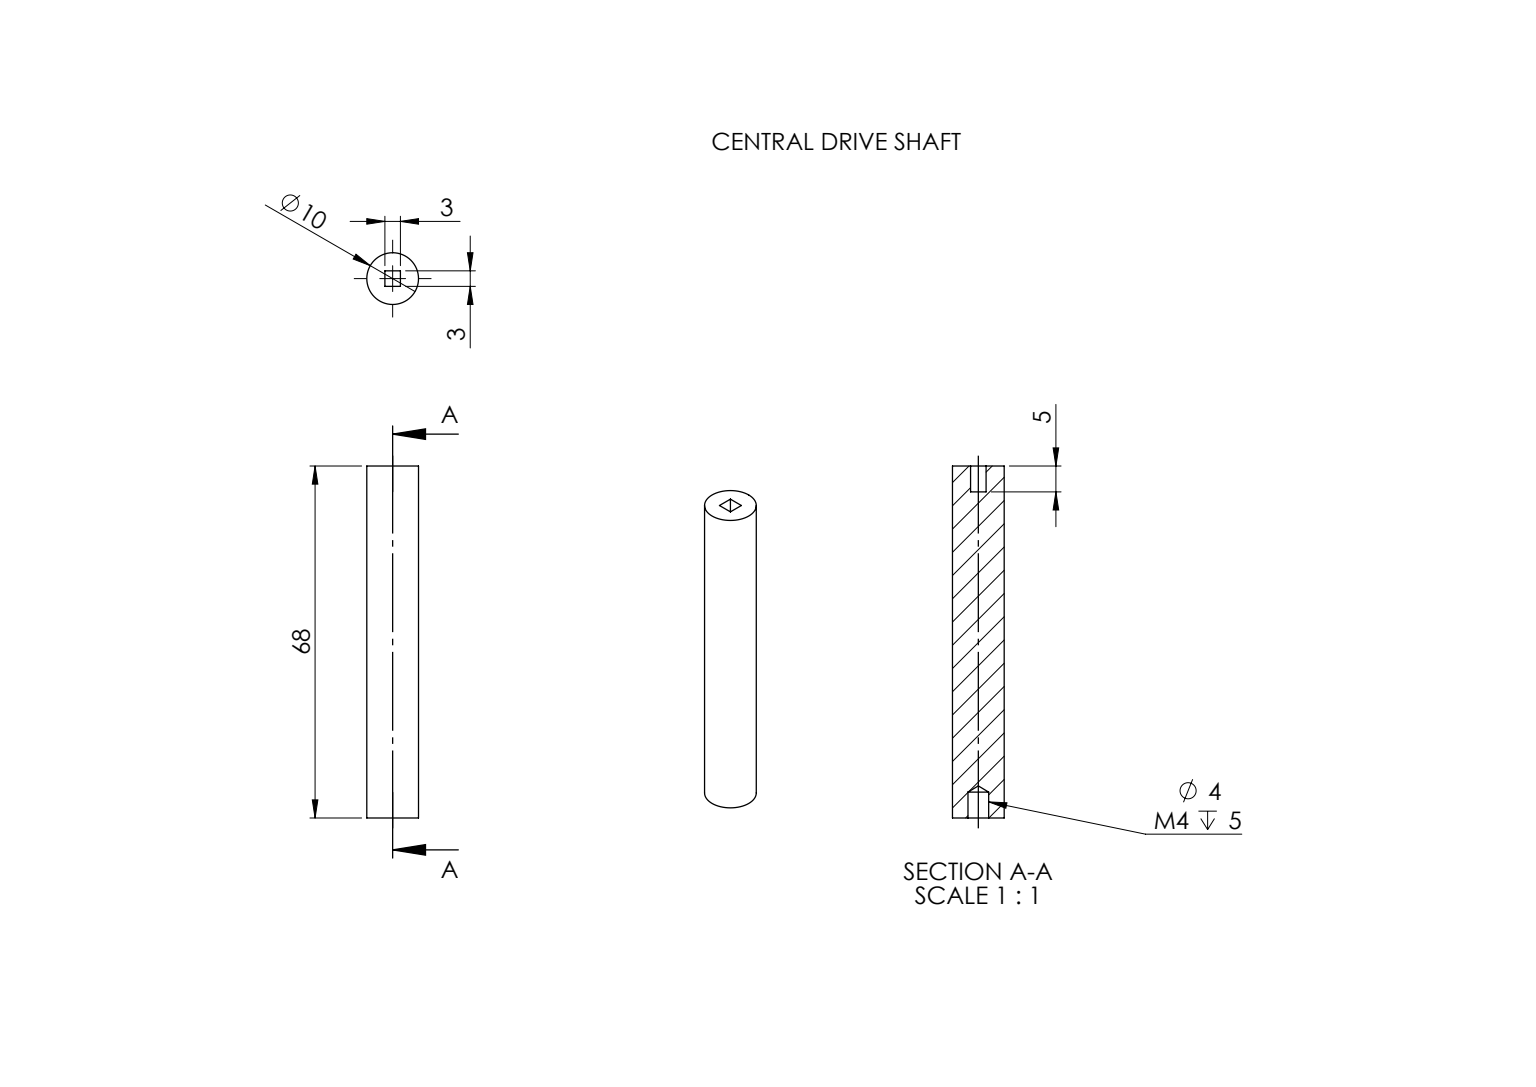
ISO-10303-21;
HEADER;
FILE_DESCRIPTION (('STEP AP214'),
    '1' );
FILE_NAME ('Central Drive Shaft.step',
    '2026-10-04T07:23:31',
    ( '' ),
    ( '' ),
    'SwSTEP 2.0',
    'SolidWorks 2026',
    '' );
FILE_SCHEMA (( 'AUTOMOTIVE_DESIGN' ));
ENDSEC;

DATA;
#2=VERTEX_POINT ( 'NONE', #10191 ) ;
#44=DIRECTION ( 'NONE',  ( 0.000000000000000000, 0.000000000000000000, -1.000000000000000000 ) ) ;
#47=ORIENTED_EDGE ( 'NONE', *, *, #865, .T. ) ;
#60=CARTESIAN_POINT ( 'NONE',  ( -1.500000000000000444, 83.00000000000000000, -1.500000000000000222 ) ) ;
#114=DIRECTION ( 'NONE',  ( 1.000000000000000000, 0.000000000000000000, -0.000000000000000000 ) ) ;
#146=DIRECTION ( 'NONE',  ( -0.000000000000000000, -1.000000000000000000, -0.000000000000000000 ) ) ;
#223=CARTESIAN_POINT ( 'NONE',  ( 0.000000000000000000, 25.00000000000000355, -2.000000000000000000 ) ) ;
#266=DIRECTION ( 'NONE',  ( 0.000000000000000000, 0.000000000000000000, -1.000000000000000000 ) ) ;
#348=DIRECTION ( 'NONE',  ( 0.000000000000000000, 0.000000000000000000, -1.000000000000000000 ) ) ;
#352=( LENGTH_UNIT ( ) NAMED_UNIT ( * ) SI_UNIT ( .MILLI., .METRE. ) );
#356=PLANE ( 'NONE',  #3904 ) ;
#359=ORIENTED_EDGE ( 'NONE', *, *, #8815, .F. ) ;
#393=ORIENTED_EDGE ( 'NONE', *, *, #10575, .T. ) ;
#405=CIRCLE ( 'NONE', #9386, 2.000000000000000000 ) ;
#454=CARTESIAN_POINT ( 'NONE',  ( 0.000000000000000000, 88.00000000000001421, 0.000000000000000000 ) ) ;
#460=CARTESIAN_POINT ( 'NONE',  ( 0.000000000000000000, 88.00000000000001421, -4.999999999999997335 ) ) ;
#485=MECHANICAL_DESIGN_GEOMETRIC_PRESENTATION_REPRESENTATION('',(#10900),#6489);
#492=VERTEX_POINT ( 'NONE', #223 ) ;
#536=DIRECTION ( 'NONE',  ( 0.000000000000000000, 1.000000000000000000, 0.000000000000000000 ) ) ;
#537=ORIENTED_EDGE ( 'NONE', *, *, #3535, .F. ) ;
#559=DIRECTION ( 'NONE',  ( 1.445602896647339163E-16, 0.000000000000000000, 1.000000000000000000 ) ) ;
#632=EDGE_LOOP ( 'NONE', ( #359, #6659, #4247, #3379 ) ) ;
#649=LINE ( 'NONE', #7380, #8128 ) ;
#650=SURFACE_STYLE_USAGE ( .BOTH. , #5631 ) ;
#693=CARTESIAN_POINT ( 'NONE',  ( -1.500000000000000444, 83.00000000000000000, -1.500000000000000222 ) ) ;
#753=CARTESIAN_POINT ( 'NONE',  ( 0.000000000000000000, 20.00000000000000355, 0.000000000000000000 ) ) ;
#771=VECTOR ( 'NONE', #10871, 1000.000000000000000 ) ;
#785=SURFACE_STYLE_FILL_AREA ( #5806 ) ;
#787=CARTESIAN_POINT ( 'NONE',  ( 0.000000000000000000, 26.20172123805511788, 0.000000000000000000 ) ) ;
#795=VERTEX_POINT ( 'NONE', #460 ) ;
#859=VERTEX_POINT ( 'NONE', #787 ) ;
#865=EDGE_CURVE ( 'NONE', #4894, #10263, #9114, .T. ) ;
#872=PLANE ( 'NONE',  #1414 ) ;
#1039=EDGE_LOOP ( 'NONE', ( #7017, #6117, #1492, #5769 ) ) ;
#1055=LINE ( 'NONE', #10332, #4311 ) ;
#1056=DIRECTION ( 'NONE',  ( -0.000000000000000000, -1.000000000000000000, -0.000000000000000000 ) ) ;
#1156=ORIENTED_EDGE ( 'NONE', *, *, #1512, .F. ) ;
#1161=CYLINDRICAL_SURFACE ( 'NONE', #5135, 2.000000000000000000 ) ;
#1178=ORIENTED_EDGE ( 'NONE', *, *, #2398, .T. ) ;
#1228=LINE ( 'NONE', #7862, #1419 ) ;
#1356=DIRECTION ( 'NONE',  ( 0.000000000000000000, 0.000000000000000000, -1.000000000000000000 ) ) ;
#1360=STYLED_ITEM ( 'NONE', ( #2425 ), #9406 ) ;
#1365=VECTOR ( 'NONE', #5254, 1000.000000000000000 ) ;
#1414=AXIS2_PLACEMENT_3D ( 'NONE', #7498, #1757, #3275 ) ;
#1419=VECTOR ( 'NONE', #2096, 1000.000000000000000 ) ;
#1443=ORIENTED_EDGE ( 'NONE', *, *, #6772, .F. ) ;
#1448=AXIS2_PLACEMENT_3D ( 'NONE', #4540, #3796, #1356 ) ;
#1468=AXIS2_PLACEMENT_3D ( 'NONE', #5195, #2673, #1693 ) ;
#1492=ORIENTED_EDGE ( 'NONE', *, *, #2347, .T. ) ;
#1499=SHAPE_REPRESENTATION_RELATIONSHIP ( 'NONE' , 'NONE' ,  #2382, #9406 ) ;
#1500=DIRECTION ( 'NONE',  ( -0.000000000000000000, -1.000000000000000000, -0.000000000000000000 ) ) ;
#1512=EDGE_CURVE ( 'NONE', #7692, #795, #8292, .T. ) ;
#1521=DIRECTION ( 'NONE',  ( 0.000000000000000000, -0.000000000000000000, 1.000000000000000000 ) ) ;
#1554=COLOUR_RGB ( '', 0.08235294, 0.09019608, 0.10196078) ;
#1588=ADVANCED_FACE ( 'NONE', ( #6010 ), #1161, .F. ) ;
#1649=PRODUCT_CONTEXT ( 'NONE', #4853, 'mechanical' ) ;
#1654=CONICAL_SURFACE ( 'NONE', #4677, 2.000000000000000000, 1.029744258676657198 ) ;
#1693=DIRECTION ( 'NONE',  ( 0.000000000000000000, 0.000000000000000000, -1.000000000000000000 ) ) ;
#1705=ORIENTED_EDGE ( 'NONE', *, *, #4329, .F. ) ;
#1712=( NAMED_UNIT ( * ) PLANE_ANGLE_UNIT ( ) SI_UNIT ( $, .RADIAN. ) );
#1719=COLOUR_RGB ( '', 0.08235294, 0.09019608, 0.10196078) ;
#1725=UNCERTAINTY_MEASURE_WITH_UNIT (LENGTH_MEASURE( 1.000000000000000082E-05 ), #9113, 'distance_accuracy_value', 'NONE');
#1739=ORIENTED_EDGE ( 'NONE', *, *, #5885, .T. ) ;
#1744=DIRECTION ( 'NONE',  ( 0.000000000000000000, 0.000000000000000000, -1.000000000000000000 ) ) ;
#1757=DIRECTION ( 'NONE',  ( -0.000000000000000000, 0.000000000000000000, 1.000000000000000000 ) ) ;
#1759=LINE ( 'NONE', #6132, #1365 ) ;
#1781=VECTOR ( 'NONE', #8968, 1000.000000000000000 ) ;
#1819=FACE_OUTER_BOUND ( 'NONE', #7522, .T. ) ;
#1843=VERTEX_POINT ( 'NONE', #7167 ) ;
#1904=CARTESIAN_POINT ( 'NONE',  ( 0.000000000000000000, 0.000000000000000000, 0.000000000000000000 ) ) ;
#1953=PRODUCT_DEFINITION_SHAPE ( 'NONE', 'NONE',  #6924 ) ;
#1990=LINE ( 'NONE', #2225, #1781 ) ;
#2005=DIRECTION ( 'NONE',  ( -0.000000000000000000, -0.000000000000000000, -1.000000000000000000 ) ) ;
#2007=CARTESIAN_POINT ( 'NONE',  ( -1.500000000000000444, 83.00000000000000000, 1.499999999999999778 ) ) ;
#2016=ORIENTED_EDGE ( 'NONE', *, *, #3973, .F. ) ;
#2018=ADVANCED_FACE ( 'NONE', ( #4526, #8756 ), #356, .T. ) ;
#2096=DIRECTION ( 'NONE',  ( 1.000000000000000000, 0.000000000000000000, 0.000000000000000000 ) ) ;
#2148=LINE ( 'NONE', #8679, #6194 ) ;
#2201=EDGE_CURVE ( 'NONE', #859, #2, #10622, .T. ) ;
#2225=CARTESIAN_POINT ( 'NONE',  ( 0.000000000000000000, 88.00000000000001421, -4.999999999999997335 ) ) ;
#2228=FACE_OUTER_BOUND ( 'NONE', #6950, .T. ) ;
#2245=SURFACE_STYLE_FILL_AREA ( #9813 ) ;
#2268=CARTESIAN_POINT ( 'NONE',  ( -1.500000000000000444, 88.00000000000001421, -1.500000000000000222 ) ) ;
#2320=FILL_AREA_STYLE_COLOUR ( '', #1554 ) ;
#2332=ORIENTED_EDGE ( 'NONE', *, *, #3800, .T. ) ;
#2347=EDGE_CURVE ( 'NONE', #6423, #4034, #2479, .T. ) ;
#2382=SHAPE_REPRESENTATION ( 'Central Drive Shaft', ( #7040 ), #8612 ) ;
#2398=EDGE_CURVE ( 'NONE', #1843, #6119, #8817, .T. ) ;
#2425=PRESENTATION_STYLE_ASSIGNMENT (( #9885 ) ) ;
#2435=CYLINDRICAL_SURFACE ( 'NONE', #8843, 4.999999999999997335 ) ;
#2460=CARTESIAN_POINT ( 'NONE',  ( 1.500000000000000000, 83.00000000000000000, 1.500000000000000000 ) ) ;
#2479=LINE ( 'NONE', #10002, #10939 ) ;
#2497=CONICAL_SURFACE ( 'NONE', #4996, 2.000000000000000000, 1.029744258676657198 ) ;
#2503=CARTESIAN_POINT ( 'NONE',  ( 0.000000000000000000, 88.00000000000001421, 0.000000000000000000 ) ) ;
#2519=FACE_OUTER_BOUND ( 'NONE', #3141, .T. ) ;
#2521=ADVANCED_FACE ( 'NONE', ( #3254 ), #10013, .T. ) ;
#2629=VECTOR ( 'NONE', #9256, 1000.000000000000000 ) ;
#2639=FACE_OUTER_BOUND ( 'NONE', #8178, .T. ) ;
#2673=DIRECTION ( 'NONE',  ( -0.000000000000000000, -1.000000000000000000, -0.000000000000000000 ) ) ;
#2736=ORIENTED_EDGE ( 'NONE', *, *, #6328, .T. ) ;
#2857=CIRCLE ( 'NONE', #4995, 4.999999999999997335 ) ;
#2884=DIRECTION ( 'NONE',  ( 0.000000000000000000, -0.000000000000000000, -1.000000000000000000 ) ) ;
#3114=CARTESIAN_POINT ( 'NONE',  ( -1.500000000000000444, 83.00000000000000000, 1.499999999999999778 ) ) ;
#3122=VECTOR ( 'NONE', #9223, 1000.000000000000000 ) ;
#3127=ORIENTED_EDGE ( 'NONE', *, *, #9759, .F. ) ;
#3141=EDGE_LOOP ( 'NONE', ( #6644, #3675, #8996 ) ) ;
#3201=DIRECTION ( 'NONE',  ( 0.000000000000000000, 0.000000000000000000, -1.000000000000000000 ) ) ;
#3254=FACE_OUTER_BOUND ( 'NONE', #632, .T. ) ;
#3275=DIRECTION ( 'NONE',  ( 1.000000000000000000, 0.000000000000000000, 0.000000000000000000 ) ) ;
#3306=FACE_OUTER_BOUND ( 'NONE', #4013, .T. ) ;
#3320=EDGE_CURVE ( 'NONE', #9769, #4894, #649, .T. ) ;
#3341=LINE ( 'NONE', #5907, #2629 ) ;
#3359=VECTOR ( 'NONE', #3900, 1000.000000000000000 ) ;
#3379=ORIENTED_EDGE ( 'NONE', *, *, #8473, .T. ) ;
#3402=ADVANCED_FACE ( 'NONE', ( #9376, #6675 ), #5136, .F. ) ;
#3416=ADVANCED_FACE ( 'NONE', ( #1819 ), #872, .T. ) ;
#3418=PLANE ( 'NONE',  #9594 ) ;
#3431=DIRECTION ( 'NONE',  ( 0.000000000000000000, 0.000000000000000000, 1.000000000000000000 ) ) ;
#3445=FACE_OUTER_BOUND ( 'NONE', #8136, .T. ) ;
#3448=CARTESIAN_POINT ( 'NONE',  ( 0.000000000000000000, 20.00000000000000355, 0.000000000000000000 ) ) ;
#3531=EDGE_LOOP ( 'NONE', ( #9699, #10736 ) ) ;
#3535=EDGE_CURVE ( 'NONE', #795, #4001, #1990, .T. ) ;
#3549=AXIS2_PLACEMENT_3D ( 'NONE', #5110, #6714, #7420 ) ;
#3621=LINE ( 'NONE', #4346, #5871 ) ;
#3627=DIRECTION ( 'NONE',  ( -0.000000000000000000, -1.000000000000000000, -0.000000000000000000 ) ) ;
#3640=ADVANCED_FACE ( 'NONE', ( #3306 ), #2435, .T. ) ;
#3641=DIRECTION ( 'NONE',  ( 0.000000000000000000, -1.000000000000000000, 0.000000000000000000 ) ) ;
#3674=ORIENTED_EDGE ( 'NONE', *, *, #10458, .F. ) ;
#3675=ORIENTED_EDGE ( 'NONE', *, *, #2201, .T. ) ;
#3774=VERTEX_POINT ( 'NONE', #9994 ) ;
#3796=DIRECTION ( 'NONE',  ( -0.000000000000000000, -1.000000000000000000, -0.000000000000000000 ) ) ;
#3800=EDGE_CURVE ( 'NONE', #3774, #10263, #4988, .T. ) ;
#3811=DIRECTION ( 'NONE',  ( 1.445602896647339163E-16, 0.000000000000000000, 1.000000000000000000 ) ) ;
#3900=DIRECTION ( 'NONE',  ( -0.000000000000000000, 1.000000000000000000, -0.000000000000000000 ) ) ;
#3904=AXIS2_PLACEMENT_3D ( 'NONE', #7105, #10470, #2884 ) ;
#3947=EDGE_LOOP ( 'NONE', ( #9642, #1156 ) ) ;
#3951=EDGE_LOOP ( 'NONE', ( #5906, #4563 ) ) ;
#3973=EDGE_CURVE ( 'NONE', #8246, #3774, #1228, .T. ) ;
#3983=CARTESIAN_POINT ( 'NONE',  ( 6.123233995736763324E-16, 20.00000000000000355, 4.999999999999997335 ) ) ;
#4001=VERTEX_POINT ( 'NONE', #7184 ) ;
#4013=EDGE_LOOP ( 'NONE', ( #1739, #8966, #1443, #537 ) ) ;
#4024=EDGE_CURVE ( 'NONE', #3774, #6423, #2148, .T. ) ;
#4034=VERTEX_POINT ( 'NONE', #2007 ) ;
#4158=CARTESIAN_POINT ( 'NONE',  ( 1.500000000000000000, 88.00000000000001421, 1.500000000000000000 ) ) ;
#4159=DIRECTION ( 'NONE',  ( -1.000000000000000000, -0.000000000000000000, -7.228014483236695816E-17 ) ) ;
#4190=SHAPE_DEFINITION_REPRESENTATION ( #1953, #2382 ) ;
#4229=VECTOR ( 'NONE', #8226, 1000.000000000000000 ) ;
#4247=ORIENTED_EDGE ( 'NONE', *, *, #4024, .T. ) ;
#4263=DIRECTION ( 'NONE',  ( -0.000000000000000000, -1.000000000000000000, -0.000000000000000000 ) ) ;
#4279=VECTOR ( 'NONE', #2005, 1000.000000000000000 ) ;
#4311=VECTOR ( 'NONE', #3641, 1000.000000000000000 ) ;
#4329=EDGE_CURVE ( 'NONE', #492, #6119, #3341, .T. ) ;
#4346=CARTESIAN_POINT ( 'NONE',  ( 2.449293598294706414E-16, 20.00000000000000355, 2.000000000000000000 ) ) ;
#4526=FACE_BOUND ( 'NONE', #3531, .T. ) ;
#4540=CARTESIAN_POINT ( 'NONE',  ( 0.000000000000000000, 20.00000000000000355, 0.000000000000000000 ) ) ;
#4563=ORIENTED_EDGE ( 'NONE', *, *, #8479, .T. ) ;
#4597=FACE_OUTER_BOUND ( 'NONE', #1039, .T. ) ;
#4606=AXIS2_PLACEMENT_3D ( 'NONE', #6774, #6652, #5062 ) ;
#4630=CIRCLE ( 'NONE', #3549, 4.999999999999997335 ) ;
#4677=AXIS2_PLACEMENT_3D ( 'NONE', #10800, #8194, #6444 ) ;
#4693=CARTESIAN_POINT ( 'NONE',  ( 0.000000000000000000, 25.00000000000000355, 0.000000000000000000 ) ) ;
#4848=CARTESIAN_POINT ( 'NONE',  ( 1.500000000000000000, 83.00000000000000000, 1.500000000000000000 ) ) ;
#4853=APPLICATION_CONTEXT ( 'automotive_design' ) ;
#4865=DIRECTION ( 'NONE',  ( -0.000000000000000000, -0.000000000000000000, -1.000000000000000000 ) ) ;
#4867=ADVANCED_FACE ( 'NONE', ( #3445 ), #5193, .T. ) ;
#4881=CARTESIAN_POINT ( 'NONE',  ( 0.000000000000000000, 20.00000000000000355, 0.000000000000000000 ) ) ;
#4893=ORIENTED_EDGE ( 'NONE', *, *, #5065, .T. ) ;
#4894=VERTEX_POINT ( 'NONE', #6070 ) ;
#4902=LINE ( 'NONE', #693, #771 ) ;
#4924=ORIENTED_EDGE ( 'NONE', *, *, #9689, .T. ) ;
#4948=AXIS2_PLACEMENT_3D ( 'NONE', #4881, #1500, #10784 ) ;
#4988=LINE ( 'NONE', #6698, #4229 ) ;
#4995=AXIS2_PLACEMENT_3D ( 'NONE', #753, #6723, #1744 ) ;
#4996=AXIS2_PLACEMENT_3D ( 'NONE', #5909, #1056, #44 ) ;
#5043=ORIENTED_EDGE ( 'NONE', *, *, #8094, .T. ) ;
#5053=ORIENTED_EDGE ( 'NONE', *, *, #8479, .F. ) ;
#5062=DIRECTION ( 'NONE',  ( 1.445602896647339163E-16, 0.000000000000000000, 1.000000000000000000 ) ) ;
#5065=EDGE_CURVE ( 'NONE', #859, #492, #9026, .T. ) ;
#5071=ADVANCED_FACE ( 'NONE', ( #2228 ), #1654, .F. ) ;
#5078=EDGE_LOOP ( 'NONE', ( #3127, #8413, #1178, #1705 ) ) ;
#5110=CARTESIAN_POINT ( 'NONE',  ( 0.000000000000000000, 20.00000000000000355, 0.000000000000000000 ) ) ;
#5135=AXIS2_PLACEMENT_3D ( 'NONE', #3448, #3627, #266 ) ;
#5136=PLANE ( 'NONE',  #6727 ) ;
#5193=CYLINDRICAL_SURFACE ( 'NONE', #7650, 4.999999999999997335 ) ;
#5195=CARTESIAN_POINT ( 'NONE',  ( 0.000000000000000000, 25.00000000000000355, 0.000000000000000000 ) ) ;
#5254=DIRECTION ( 'NONE',  ( -1.000000000000000000, -0.000000000000000000, -7.228014483236695816E-17 ) ) ;
#5419=DIRECTION ( 'NONE',  ( 0.000000000000000000, 0.000000000000000000, -1.000000000000000000 ) ) ;
#5519=ADVANCED_FACE ( 'NONE', ( #2519 ), #2497, .F. ) ;
#5601=MECHANICAL_DESIGN_GEOMETRIC_PRESENTATION_REPRESENTATION('',(#1360),#8410);
#5606=UNCERTAINTY_MEASURE_WITH_UNIT (LENGTH_MEASURE( 1.000000000000000082E-05 ), #352, 'distance_accuracy_value', 'NONE');
#5631=SURFACE_SIDE_STYLE ('',( #2245 ) ) ;
#5749=ORIENTED_EDGE ( 'NONE', *, *, #3973, .T. ) ;
#5769=ORIENTED_EDGE ( 'NONE', *, *, #10458, .T. ) ;
#5806=FILL_AREA_STYLE ('',( #2320 ) ) ;
#5818=ORIENTED_EDGE ( 'NONE', *, *, #2347, .F. ) ;
#5869=CARTESIAN_POINT ( 'NONE',  ( 2.449293598294706414E-16, 25.00000000000000355, 2.000000000000000000 ) ) ;
#5870=EDGE_CURVE ( 'NONE', #492, #2, #10108, .T. ) ;
#5871=VECTOR ( 'NONE', #146, 1000.000000000000000 ) ;
#5885=EDGE_CURVE ( 'NONE', #795, #7692, #9412, .T. ) ;
#5903=DIRECTION ( 'NONE',  ( 0.000000000000000000, -1.000000000000000000, 0.000000000000000000 ) ) ;
#5906=ORIENTED_EDGE ( 'NONE', *, *, #6772, .T. ) ;
#5907=CARTESIAN_POINT ( 'NONE',  ( 0.000000000000000000, 20.00000000000000355, -2.000000000000000000 ) ) ;
#5909=CARTESIAN_POINT ( 'NONE',  ( 0.000000000000000000, 25.00000000000000355, 0.000000000000000000 ) ) ;
#5925=DIRECTION ( 'NONE',  ( 1.049727191138620421E-16, -0.5150380749100518241, 0.8571673007021137769 ) ) ;
#6007=DIRECTION ( 'NONE',  ( 0.000000000000000000, -1.000000000000000000, 0.000000000000000000 ) ) ;
#6010=FACE_OUTER_BOUND ( 'NONE', #5078, .T. ) ;
#6070=CARTESIAN_POINT ( 'NONE',  ( -1.500000000000000444, 88.00000000000001421, -1.500000000000000222 ) ) ;
#6104=PRODUCT ( 'Central Drive Shaft', 'Central Drive Shaft', '', ( #1649 ) ) ;
#6117=ORIENTED_EDGE ( 'NONE', *, *, #8473, .F. ) ;
#6119=VERTEX_POINT ( 'NONE', #7680 ) ;
#6131=ORIENTED_EDGE ( 'NONE', *, *, #5870, .F. ) ;
#6132=CARTESIAN_POINT ( 'NONE',  ( -1.500000000000000444, 88.00000000000001421, 1.499999999999999778 ) ) ;
#6194=VECTOR ( 'NONE', #3811, 1000.000000000000000 ) ;
#6239=CARTESIAN_POINT ( 'NONE',  ( -1.500000000000000444, 83.00000000000000000, -1.500000000000000222 ) ) ;
#6253=CARTESIAN_POINT ( 'NONE',  ( -1.500000000000000444, 83.00000000000000000, 1.499999999999999778 ) ) ;
#6304=LINE ( 'NONE', #10446, #4279 ) ;
#6328=EDGE_CURVE ( 'NONE', #4034, #8246, #6304, .T. ) ;
#6379=( NAMED_UNIT ( * ) PLANE_ANGLE_UNIT ( ) SI_UNIT ( $, .RADIAN. ) );
#6408=CARTESIAN_POINT ( 'NONE',  ( 0.000000000000000000, 83.00000000000000000, 0.000000000000000000 ) ) ;
#6423=VERTEX_POINT ( 'NONE', #2460 ) ;
#6444=DIRECTION ( 'NONE',  ( 0.000000000000000000, 0.000000000000000000, -1.000000000000000000 ) ) ;
#6461=FILL_AREA_STYLE_COLOUR ( '', #1719 ) ;
#6489=( GEOMETRIC_REPRESENTATION_CONTEXT ( 3 ) GLOBAL_UNCERTAINTY_ASSIGNED_CONTEXT ( ( #9021 ) ) GLOBAL_UNIT_ASSIGNED_CONTEXT ( ( #10704, #10758, #10266 ) ) REPRESENTATION_CONTEXT ( 'NONE', 'WORKASPACE' ) );
#6517=PRODUCT_DEFINITION_FORMATION_WITH_SPECIFIED_SOURCE ( 'ANY', '', #6104, .NOT_KNOWN. ) ;
#6539=AXIS2_PLACEMENT_3D ( 'NONE', #454, #9524, #348 ) ;
#6563=AXIS2_PLACEMENT_3D ( 'NONE', #10169, #4263, #5419 ) ;
#6578=ORIENTED_EDGE ( 'NONE', *, *, #3320, .T. ) ;
#6644=ORIENTED_EDGE ( 'NONE', *, *, #5065, .F. ) ;
#6652=DIRECTION ( 'NONE',  ( -1.000000000000000000, 0.000000000000000000, 1.445602896647339163E-16 ) ) ;
#6659=ORIENTED_EDGE ( 'NONE', *, *, #3800, .F. ) ;
#6675=FACE_BOUND ( 'NONE', #7451, .T. ) ;
#6676=DIRECTION ( 'NONE',  ( -0.000000000000000000, 1.000000000000000000, -0.000000000000000000 ) ) ;
#6698=CARTESIAN_POINT ( 'NONE',  ( 1.499999999999999556, 83.00000000000000000, -1.500000000000000222 ) ) ;
#6714=DIRECTION ( 'NONE',  ( 0.000000000000000000, -1.000000000000000000, 0.000000000000000000 ) ) ;
#6723=DIRECTION ( 'NONE',  ( 0.000000000000000000, -1.000000000000000000, 0.000000000000000000 ) ) ;
#6727=AXIS2_PLACEMENT_3D ( 'NONE', #8486, #5903, #9252 ) ;
#6750=ORIENTED_EDGE ( 'NONE', *, *, #5870, .T. ) ;
#6755=CIRCLE ( 'NONE', #1448, 2.000000000000000000 ) ;
#6771=AXIS2_PLACEMENT_3D ( 'NONE', #2503, #7716, #6962 ) ;
#6772=EDGE_CURVE ( 'NONE', #4001, #7375, #2857, .T. ) ;
#6774=CARTESIAN_POINT ( 'NONE',  ( 1.499999999999999556, 83.00000000000000000, -1.500000000000000222 ) ) ;
#6836=CARTESIAN_POINT ( 'NONE',  ( 0.000000000000000000, 88.00000000000001421, 0.000000000000000000 ) ) ;
#6899=DIRECTION ( 'NONE',  ( 0.000000000000000000, 0.000000000000000000, -1.000000000000000000 ) ) ;
#6924=PRODUCT_DEFINITION ( 'UNKNOWN', '', #6517, #8802 ) ;
#6949=EDGE_CURVE ( 'NONE', #2, #1843, #3621, .T. ) ;
#6950=EDGE_LOOP ( 'NONE', ( #10094, #4893, #6750 ) ) ;
#6962=DIRECTION ( 'NONE',  ( 0.000000000000000000, 0.000000000000000000, -1.000000000000000000 ) ) ;
#6970=VECTOR ( 'NONE', #8240, 1000.000000000000114 ) ;
#6988=ORIENTED_EDGE ( 'NONE', *, *, #1512, .T. ) ;
#6989=ORIENTED_EDGE ( 'NONE', *, *, #6328, .F. ) ;
#7017=ORIENTED_EDGE ( 'NONE', *, *, #10575, .F. ) ;
#7040=AXIS2_PLACEMENT_3D ( 'NONE', #1904, #3431, #7048 ) ;
#7048=DIRECTION ( 'NONE',  ( 1.000000000000000000, 0.000000000000000000, 0.000000000000000000 ) ) ;
#7071=ORIENTED_EDGE ( 'NONE', *, *, #6949, .F. ) ;
#7105=CARTESIAN_POINT ( 'NONE',  ( 0.000000000000000000, 20.00000000000000355, 0.000000000000000000 ) ) ;
#7130=AXIS2_PLACEMENT_3D ( 'NONE', #6253, #9557, #7791 ) ;
#7167=CARTESIAN_POINT ( 'NONE',  ( 2.449293598294706414E-16, 20.00000000000000355, 2.000000000000000000 ) ) ;
#7184=CARTESIAN_POINT ( 'NONE',  ( 0.000000000000000000, 20.00000000000000355, -4.999999999999997335 ) ) ;
#7196=ADVANCED_FACE ( 'NONE', ( #2639 ), #3418, .T. ) ;
#7322=FACE_OUTER_BOUND ( 'NONE', #8137, .T. ) ;
#7375=VERTEX_POINT ( 'NONE', #3983 ) ;
#7380=CARTESIAN_POINT ( 'NONE',  ( -1.500000000000000444, 88.00000000000001421, -1.500000000000000222 ) ) ;
#7414=DIRECTION ( 'NONE',  ( 0.000000000000000000, -1.000000000000000000, 0.000000000000000000 ) ) ;
#7420=DIRECTION ( 'NONE',  ( 0.000000000000000000, 0.000000000000000000, -1.000000000000000000 ) ) ;
#7451=EDGE_LOOP ( 'NONE', ( #10021, #393, #6578, #47 ) ) ;
#7498=CARTESIAN_POINT ( 'NONE',  ( -1.500000000000000444, 83.00000000000000000, -1.500000000000000222 ) ) ;
#7522=EDGE_LOOP ( 'NONE', ( #8899, #9738, #5749, #2332 ) ) ;
#7567=DIRECTION ( 'NONE',  ( -0.000000000000000000, 0.000000000000000000, -1.000000000000000000 ) ) ;
#7650=AXIS2_PLACEMENT_3D ( 'NONE', #6836, #6007, #6899 ) ;
#7672=ADVANCED_FACE ( 'NONE', ( #4597 ), #10490, .T. ) ;
#7680=CARTESIAN_POINT ( 'NONE',  ( 0.000000000000000000, 20.00000000000000355, -2.000000000000000000 ) ) ;
#7692=VERTEX_POINT ( 'NONE', #8775 ) ;
#7716=DIRECTION ( 'NONE',  ( 0.000000000000000000, -1.000000000000000000, 0.000000000000000000 ) ) ;
#7791=DIRECTION ( 'NONE',  ( -1.000000000000000000, 0.000000000000000000, -7.228014483236695816E-17 ) ) ;
#7798=CARTESIAN_POINT ( 'NONE',  ( 1.499999999999999556, 88.00000000000001421, -1.500000000000000222 ) ) ;
#7804=EDGE_CURVE ( 'NONE', #7692, #7375, #1055, .T. ) ;
#7813=AXIS2_PLACEMENT_3D ( 'NONE', #6408, #536, #1521 ) ;
#7862=CARTESIAN_POINT ( 'NONE',  ( -1.500000000000000444, 83.00000000000000000, -1.500000000000000222 ) ) ;
#7952=CYLINDRICAL_SURFACE ( 'NONE', #6563, 2.000000000000000000 ) ;
#8094=EDGE_CURVE ( 'NONE', #8246, #4894, #4902, .T. ) ;
#8128=VECTOR ( 'NONE', #4865, 1000.000000000000000 ) ;
#8136=EDGE_LOOP ( 'NONE', ( #10493, #6988, #10509, #5053 ) ) ;
#8137=EDGE_LOOP ( 'NONE', ( #9423, #2016, #6989, #5818 ) ) ;
#8145=CARTESIAN_POINT ( 'NONE',  ( 0.000000000000000000, 25.00000000000000355, -2.000000000000000000 ) ) ;
#8178=EDGE_LOOP ( 'NONE', ( #10151, #3674, #2736, #5043 ) ) ;
#8194=DIRECTION ( 'NONE',  ( -0.000000000000000000, -1.000000000000000000, -0.000000000000000000 ) ) ;
#8226=DIRECTION ( 'NONE',  ( -0.000000000000000000, 1.000000000000000000, -0.000000000000000000 ) ) ;
#8240=DIRECTION ( 'NONE',  ( 0.000000000000000000, -0.5150380749100518241, -0.8571673007021137769 ) ) ;
#8246=VERTEX_POINT ( 'NONE', #6239 ) ;
#8292=CIRCLE ( 'NONE', #6539, 4.999999999999997335 ) ;
#8343=( NAMED_UNIT ( * ) SI_UNIT ( $, .STERADIAN. ) SOLID_ANGLE_UNIT ( ) );
#8410=( GEOMETRIC_REPRESENTATION_CONTEXT ( 3 ) GLOBAL_UNCERTAINTY_ASSIGNED_CONTEXT ( ( #1725 ) ) GLOBAL_UNIT_ASSIGNED_CONTEXT ( ( #9113, #1712, #8343 ) ) REPRESENTATION_CONTEXT ( 'NONE', 'WORKASPACE' ) );
#8413=ORIENTED_EDGE ( 'NONE', *, *, #6949, .T. ) ;
#8452=ORIENTED_EDGE ( 'NONE', *, *, #4329, .T. ) ;
#8473=EDGE_CURVE ( 'NONE', #6423, #9073, #9027, .T. ) ;
#8479=EDGE_CURVE ( 'NONE', #7375, #4001, #4630, .T. ) ;
#8486=CARTESIAN_POINT ( 'NONE',  ( 0.000000000000000000, 88.00000000000001421, 0.000000000000000000 ) ) ;
#8579=APPLICATION_CONTEXT ( 'automotive_design' ) ;
#8598=VECTOR ( 'NONE', #6676, 1000.000000000000000 ) ;
#8612=( GEOMETRIC_REPRESENTATION_CONTEXT ( 3 ) GLOBAL_UNCERTAINTY_ASSIGNED_CONTEXT ( ( #5606 ) ) GLOBAL_UNIT_ASSIGNED_CONTEXT ( ( #352, #6379, #8906 ) ) REPRESENTATION_CONTEXT ( 'NONE', 'WORKASPACE' ) );
#8679=CARTESIAN_POINT ( 'NONE',  ( 1.499999999999999556, 83.00000000000000000, -1.500000000000000222 ) ) ;
#8756=FACE_OUTER_BOUND ( 'NONE', #3951, .T. ) ;
#8775=CARTESIAN_POINT ( 'NONE',  ( 6.123233995736763324E-16, 88.00000000000001421, 4.999999999999997335 ) ) ;
#8802=PRODUCT_DEFINITION_CONTEXT ( 'detailed design', #8579, 'design' ) ;
#8815=EDGE_CURVE ( 'NONE', #10263, #9073, #10621, .T. ) ;
#8817=CIRCLE ( 'NONE', #4948, 2.000000000000000000 ) ;
#8843=AXIS2_PLACEMENT_3D ( 'NONE', #10795, #7414, #3201 ) ;
#8899=ORIENTED_EDGE ( 'NONE', *, *, #865, .F. ) ;
#8906=( NAMED_UNIT ( * ) SI_UNIT ( $, .STERADIAN. ) SOLID_ANGLE_UNIT ( ) );
#8966=ORIENTED_EDGE ( 'NONE', *, *, #7804, .T. ) ;
#8968=DIRECTION ( 'NONE',  ( 0.000000000000000000, -1.000000000000000000, 0.000000000000000000 ) ) ;
#8989=PRESENTATION_STYLE_ASSIGNMENT (( #650 ) ) ;
#8996=ORIENTED_EDGE ( 'NONE', *, *, #9759, .T. ) ;
#9021=UNCERTAINTY_MEASURE_WITH_UNIT (LENGTH_MEASURE( 1.000000000000000082E-05 ), #10704, 'distance_accuracy_value', 'NONE');
#9026=LINE ( 'NONE', #8145, #6970 ) ;
#9027=LINE ( 'NONE', #4848, #3359 ) ;
#9073=VERTEX_POINT ( 'NONE', #4158 ) ;
#9092=PLANE ( 'NONE',  #7813 ) ;
#9113=( LENGTH_UNIT ( ) NAMED_UNIT ( * ) SI_UNIT ( .MILLI., .METRE. ) );
#9114=LINE ( 'NONE', #2268, #3122 ) ;
#9199=ADVANCED_FACE ( 'NONE', ( #10540 ), #7952, .F. ) ;
#9223=DIRECTION ( 'NONE',  ( 1.000000000000000000, 0.000000000000000000, 0.000000000000000000 ) ) ;
#9252=DIRECTION ( 'NONE',  ( 0.000000000000000000, -0.000000000000000000, -1.000000000000000000 ) ) ;
#9256=DIRECTION ( 'NONE',  ( -0.000000000000000000, -1.000000000000000000, -0.000000000000000000 ) ) ;
#9270=SURFACE_SIDE_STYLE ('',( #785 ) ) ;
#9376=FACE_OUTER_BOUND ( 'NONE', #3947, .T. ) ;
#9382=ADVANCED_FACE ( 'NONE', ( #7322 ), #9092, .T. ) ;
#9386=AXIS2_PLACEMENT_3D ( 'NONE', #4693, #10582, #10740 ) ;
#9406=ADVANCED_BREP_SHAPE_REPRESENTATION ( '', ( #10557, #7040 ), #8612 ) ;
#9412=CIRCLE ( 'NONE', #6771, 4.999999999999997335 ) ;
#9423=ORIENTED_EDGE ( 'NONE', *, *, #4024, .F. ) ;
#9494=CLOSED_SHELL ( 'NONE', ( #5519, #1588, #3640, #3402, #4867, #2018, #9199, #5071, #2521, #7672, #7196, #3416, #9382 ) ) ;
#9524=DIRECTION ( 'NONE',  ( 0.000000000000000000, -1.000000000000000000, 0.000000000000000000 ) ) ;
#9557=DIRECTION ( 'NONE',  ( 7.228014483236695816E-17, 0.000000000000000000, -1.000000000000000000 ) ) ;
#9561=VECTOR ( 'NONE', #559, 1000.000000000000000 ) ;
#9594=AXIS2_PLACEMENT_3D ( 'NONE', #60, #114, #7567 ) ;
#9642=ORIENTED_EDGE ( 'NONE', *, *, #5885, .F. ) ;
#9689=EDGE_CURVE ( 'NONE', #6119, #1843, #6755, .T. ) ;
#9699=ORIENTED_EDGE ( 'NONE', *, *, #9689, .F. ) ;
#9738=ORIENTED_EDGE ( 'NONE', *, *, #8094, .F. ) ;
#9759=EDGE_CURVE ( 'NONE', #2, #492, #405, .T. ) ;
#9769=VERTEX_POINT ( 'NONE', #9800 ) ;
#9800=CARTESIAN_POINT ( 'NONE',  ( -1.500000000000000444, 88.00000000000001421, 1.499999999999999778 ) ) ;
#9813=FILL_AREA_STYLE ('',( #6461 ) ) ;
#9885=SURFACE_STYLE_USAGE ( .BOTH. , #9270 ) ;
#9978=EDGE_LOOP ( 'NONE', ( #7071, #6131, #8452, #4924 ) ) ;
#9979=LINE ( 'NONE', #3114, #8598 ) ;
#9994=CARTESIAN_POINT ( 'NONE',  ( 1.499999999999999556, 83.00000000000000000, -1.500000000000000222 ) ) ;
#10002=CARTESIAN_POINT ( 'NONE',  ( -1.500000000000000444, 83.00000000000000000, 1.499999999999999778 ) ) ;
#10013=PLANE ( 'NONE',  #4606 ) ;
#10021=ORIENTED_EDGE ( 'NONE', *, *, #8815, .T. ) ;
#10094=ORIENTED_EDGE ( 'NONE', *, *, #2201, .F. ) ;
#10108=CIRCLE ( 'NONE', #1468, 2.000000000000000000 ) ;
#10151=ORIENTED_EDGE ( 'NONE', *, *, #3320, .F. ) ;
#10169=CARTESIAN_POINT ( 'NONE',  ( 0.000000000000000000, 20.00000000000000355, 0.000000000000000000 ) ) ;
#10191=CARTESIAN_POINT ( 'NONE',  ( 2.449293598294706414E-16, 25.00000000000000355, 2.000000000000000000 ) ) ;
#10228=VECTOR ( 'NONE', #5925, 1000.000000000000114 ) ;
#10263=VERTEX_POINT ( 'NONE', #7798 ) ;
#10266=( NAMED_UNIT ( * ) SI_UNIT ( $, .STERADIAN. ) SOLID_ANGLE_UNIT ( ) );
#10332=CARTESIAN_POINT ( 'NONE',  ( 6.123233995736763324E-16, 88.00000000000001421, 4.999999999999997335 ) ) ;
#10446=CARTESIAN_POINT ( 'NONE',  ( -1.500000000000000444, 83.00000000000000000, -1.500000000000000222 ) ) ;
#10458=EDGE_CURVE ( 'NONE', #4034, #9769, #9979, .T. ) ;
#10470=DIRECTION ( 'NONE',  ( 0.000000000000000000, -1.000000000000000000, 0.000000000000000000 ) ) ;
#10490=PLANE ( 'NONE',  #7130 ) ;
#10493=ORIENTED_EDGE ( 'NONE', *, *, #7804, .F. ) ;
#10509=ORIENTED_EDGE ( 'NONE', *, *, #3535, .T. ) ;
#10540=FACE_OUTER_BOUND ( 'NONE', #9978, .T. ) ;
#10557=MANIFOLD_SOLID_BREP ( 'Cavity1', #9494 ) ;
#10575=EDGE_CURVE ( 'NONE', #9073, #9769, #1759, .T. ) ;
#10582=DIRECTION ( 'NONE',  ( -0.000000000000000000, -1.000000000000000000, -0.000000000000000000 ) ) ;
#10621=LINE ( 'NONE', #10678, #9561 ) ;
#10622=LINE ( 'NONE', #5869, #10228 ) ;
#10678=CARTESIAN_POINT ( 'NONE',  ( 1.499999999999999556, 88.00000000000001421, -1.500000000000000222 ) ) ;
#10704=( LENGTH_UNIT ( ) NAMED_UNIT ( * ) SI_UNIT ( .MILLI., .METRE. ) );
#10736=ORIENTED_EDGE ( 'NONE', *, *, #2398, .F. ) ;
#10740=DIRECTION ( 'NONE',  ( 0.000000000000000000, 0.000000000000000000, -1.000000000000000000 ) ) ;
#10758=( NAMED_UNIT ( * ) PLANE_ANGLE_UNIT ( ) SI_UNIT ( $, .RADIAN. ) );
#10784=DIRECTION ( 'NONE',  ( 0.000000000000000000, 0.000000000000000000, -1.000000000000000000 ) ) ;
#10795=CARTESIAN_POINT ( 'NONE',  ( 0.000000000000000000, 88.00000000000001421, 0.000000000000000000 ) ) ;
#10800=CARTESIAN_POINT ( 'NONE',  ( 0.000000000000000000, 25.00000000000000355, 0.000000000000000000 ) ) ;
#10871=DIRECTION ( 'NONE',  ( -0.000000000000000000, 1.000000000000000000, -0.000000000000000000 ) ) ;
#10900=STYLED_ITEM ( 'NONE', ( #8989 ), #10557 ) ;
#10939=VECTOR ( 'NONE', #4159, 1000.000000000000000 ) ;
ENDSEC;
END-ISO-10303-21;
